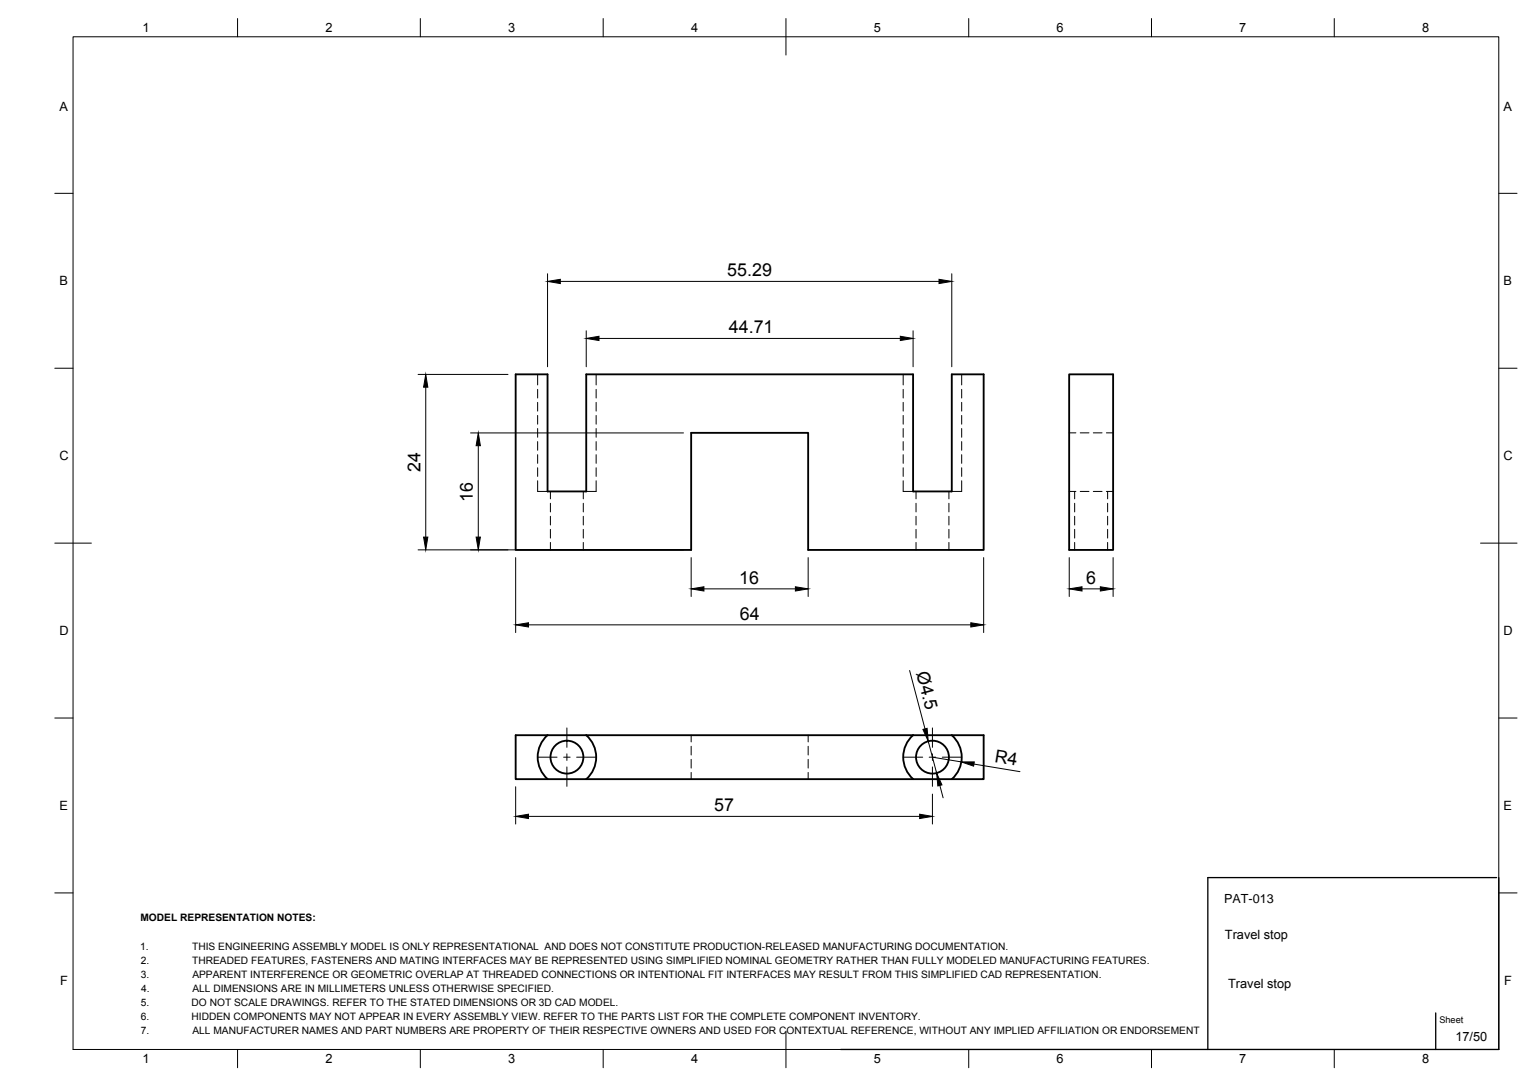
ISO-10303-21;
HEADER;
/* Generated by software containing ST-Developer
 * from STEP Tools, Inc. (www.steptools.com) 
 */

FILE_DESCRIPTION(
/* description */ ('Belt-driven linear axis on 2020 extrusion'),
/* implementation_level */ '2;1');

FILE_NAME(
/* name */ 'Travel stop.step',
/* time_stamp */ '2026-10-28T03:26:09-07:00',
/* author */ (''),
/* organization */ (''),
/* preprocessor_version */ 'ST-DEVELOPER v20.2',
/* originating_system */ 'Autodesk Translation Framework v15.17.0.0',
/* authorisation */ '');

FILE_SCHEMA (('AUTOMOTIVE_DESIGN { 1 0 10303 214 3 1 1 }'));
ENDSEC;

DATA;
#10=MECHANICAL_DESIGN_GEOMETRIC_PRESENTATION_REPRESENTATION('',(#624),#20096);
#530=SHAPE_REPRESENTATION_RELATIONSHIP('SRR','None',#20326,#576);
#576=ADVANCED_BREP_SHAPE_REPRESENTATION('',(#680),#20057);
#624=STYLED_ITEM('',(#20636),#680);
#680=MANIFOLD_SOLID_BREP('Body1',#10937);
#796=FACE_BOUND('',#2127,.T.);
#797=FACE_BOUND('',#2131,.T.);
#798=FACE_BOUND('',#2143,.T.);
#799=FACE_BOUND('',#2145,.T.);
#977=PLANE('',#11857);
#978=PLANE('',#11865);
#979=PLANE('',#11867);
#980=PLANE('',#11868);
#981=PLANE('',#11869);
#982=PLANE('',#11870);
#983=PLANE('',#11875);
#984=PLANE('',#11876);
#985=PLANE('',#11877);
#986=PLANE('',#11878);
#987=PLANE('',#11879);
#988=PLANE('',#11880);
#989=PLANE('',#11881);
#990=PLANE('',#11882);
#1424=FACE_OUTER_BOUND('',#2124,.T.);
#1425=FACE_OUTER_BOUND('',#2125,.T.);
#1426=FACE_OUTER_BOUND('',#2126,.T.);
#1427=FACE_OUTER_BOUND('',#2128,.T.);
#1428=FACE_OUTER_BOUND('',#2129,.T.);
#1429=FACE_OUTER_BOUND('',#2130,.T.);
#1430=FACE_OUTER_BOUND('',#2132,.T.);
#1431=FACE_OUTER_BOUND('',#2133,.T.);
#1432=FACE_OUTER_BOUND('',#2134,.T.);
#1433=FACE_OUTER_BOUND('',#2135,.T.);
#1434=FACE_OUTER_BOUND('',#2136,.T.);
#1435=FACE_OUTER_BOUND('',#2137,.T.);
#1436=FACE_OUTER_BOUND('',#2138,.T.);
#1437=FACE_OUTER_BOUND('',#2139,.T.);
#1438=FACE_OUTER_BOUND('',#2140,.T.);
#1439=FACE_OUTER_BOUND('',#2141,.T.);
#1440=FACE_OUTER_BOUND('',#2142,.T.);
#1441=FACE_OUTER_BOUND('',#2144,.T.);
#1442=FACE_OUTER_BOUND('',#2146,.T.);
#1443=FACE_OUTER_BOUND('',#2147,.T.);
#2124=EDGE_LOOP('',(#8009,#8010,#8011,#8012));
#2125=EDGE_LOOP('',(#8013,#8014,#8015,#8016));
#2126=EDGE_LOOP('',(#8017,#8018,#8019,#8020));
#2127=EDGE_LOOP('',(#8021));
#2128=EDGE_LOOP('',(#8022,#8023,#8024,#8025));
#2129=EDGE_LOOP('',(#8026,#8027,#8028,#8029));
#2130=EDGE_LOOP('',(#8030,#8031,#8032,#8033));
#2131=EDGE_LOOP('',(#8034));
#2132=EDGE_LOOP('',(#8035,#8036,#8037,#8038,#8039,#8040,#8041,#8042,#8043,
#8044,#8045,#8046,#8047,#8048,#8049,#8050));
#2133=EDGE_LOOP('',(#8051,#8052,#8053,#8054));
#2134=EDGE_LOOP('',(#8055,#8056,#8057,#8058));
#2135=EDGE_LOOP('',(#8059,#8060,#8061,#8062));
#2136=EDGE_LOOP('',(#8063,#8064,#8065,#8066));
#2137=EDGE_LOOP('',(#8067,#8068,#8069,#8070));
#2138=EDGE_LOOP('',(#8071,#8072,#8073,#8074));
#2139=EDGE_LOOP('',(#8075,#8076,#8077,#8078));
#2140=EDGE_LOOP('',(#8079,#8080,#8081,#8082));
#2141=EDGE_LOOP('',(#8083,#8084,#8085,#8086,#8087,#8088,#8089,#8090,#8091,
#8092,#8093,#8094,#8095,#8096,#8097,#8098));
#2142=EDGE_LOOP('',(#8099,#8100,#8101,#8102));
#2143=EDGE_LOOP('',(#8103));
#2144=EDGE_LOOP('',(#8104,#8105,#8106,#8107));
#2145=EDGE_LOOP('',(#8108));
#2146=EDGE_LOOP('',(#8109,#8110,#8111,#8112));
#2147=EDGE_LOOP('',(#8113,#8114,#8115,#8116));
#2871=LINE('',#17054,#3728);
#2872=LINE('',#17058,#3729);
#2873=LINE('',#17063,#3730);
#2874=LINE('',#17067,#3731);
#2875=LINE('',#17070,#3732);
#2876=LINE('',#17071,#3733);
#2877=LINE('',#17077,#3734);
#2878=LINE('',#17081,#3735);
#2879=LINE('',#17086,#3736);
#2880=LINE('',#17090,#3737);
#2881=LINE('',#17093,#3738);
#2882=LINE('',#17094,#3739);
#2883=LINE('',#17099,#3740);
#2884=LINE('',#17101,#3741);
#2885=LINE('',#17103,#3742);
#2886=LINE('',#17105,#3743);
#2887=LINE('',#17107,#3744);
#2888=LINE('',#17109,#3745);
#2889=LINE('',#17111,#3746);
#2890=LINE('',#17113,#3747);
#2891=LINE('',#17114,#3748);
#2892=LINE('',#17115,#3749);
#2893=LINE('',#17118,#3750);
#2894=LINE('',#17119,#3751);
#2895=LINE('',#17122,#3752);
#2896=LINE('',#17123,#3753);
#2897=LINE('',#17125,#3754);
#2898=LINE('',#17129,#3755);
#2899=LINE('',#17133,#3756);
#2900=LINE('',#17136,#3757);
#2901=LINE('',#17138,#3758);
#2902=LINE('',#17139,#3759);
#2903=LINE('',#17142,#3760);
#2904=LINE('',#17144,#3761);
#2905=LINE('',#17145,#3762);
#2906=LINE('',#17147,#3763);
#2907=LINE('',#17150,#3764);
#2908=LINE('',#17151,#3765);
#2909=LINE('',#17153,#3766);
#2910=LINE('',#17154,#3767);
#2911=LINE('',#17156,#3768);
#2912=LINE('',#17158,#3769);
#3728=VECTOR('',#13715,1.);
#3729=VECTOR('',#13718,1.);
#3730=VECTOR('',#13723,1.);
#3731=VECTOR('',#13726,1.);
#3732=VECTOR('',#13731,1.);
#3733=VECTOR('',#13732,1.);
#3734=VECTOR('',#13737,1.);
#3735=VECTOR('',#13740,1.);
#3736=VECTOR('',#13745,1.);
#3737=VECTOR('',#13748,1.);
#3738=VECTOR('',#13753,1.);
#3739=VECTOR('',#13754,1.);
#3740=VECTOR('',#13759,1.);
#3741=VECTOR('',#13760,1.);
#3742=VECTOR('',#13761,1.);
#3743=VECTOR('',#13762,1.);
#3744=VECTOR('',#13763,1.);
#3745=VECTOR('',#13764,1.);
#3746=VECTOR('',#13765,1.);
#3747=VECTOR('',#13766,1.);
#3748=VECTOR('',#13767,1.);
#3749=VECTOR('',#13768,1.);
#3750=VECTOR('',#13771,1.);
#3751=VECTOR('',#13772,1.);
#3752=VECTOR('',#13775,1.);
#3753=VECTOR('',#13776,1.);
#3754=VECTOR('',#13779,1.);
#3755=VECTOR('',#13784,0.225);
#3756=VECTOR('',#13789,0.225);
#3757=VECTOR('',#13792,1.);
#3758=VECTOR('',#13793,1.);
#3759=VECTOR('',#13794,1.);
#3760=VECTOR('',#13797,1.);
#3761=VECTOR('',#13798,1.);
#3762=VECTOR('',#13799,1.);
#3763=VECTOR('',#13802,1.);
#3764=VECTOR('',#13805,1.);
#3765=VECTOR('',#13806,1.);
#3766=VECTOR('',#13807,1.);
#3767=VECTOR('',#13808,1.);
#3768=VECTOR('',#13811,1.);
#3769=VECTOR('',#13814,1.);
#4551=CIRCLE('',#11852,0.4);
#4552=CIRCLE('',#11853,0.4);
#4553=CIRCLE('',#11855,0.4);
#4554=CIRCLE('',#11856,0.4);
#4555=CIRCLE('',#11858,0.225);
#4556=CIRCLE('',#11860,0.4);
#4557=CIRCLE('',#11861,0.4);
#4558=CIRCLE('',#11863,0.4);
#4559=CIRCLE('',#11864,0.4);
#4560=CIRCLE('',#11866,0.225);
#4561=CIRCLE('',#11872,0.225);
#4562=CIRCLE('',#11874,0.225);
#5144=VERTEX_POINT('',#17052);
#5145=VERTEX_POINT('',#17053);
#5146=VERTEX_POINT('',#17055);
#5147=VERTEX_POINT('',#17057);
#5148=VERTEX_POINT('',#17061);
#5149=VERTEX_POINT('',#17062);
#5150=VERTEX_POINT('',#17064);
#5151=VERTEX_POINT('',#17066);
#5152=VERTEX_POINT('',#17072);
#5153=VERTEX_POINT('',#17075);
#5154=VERTEX_POINT('',#17076);
#5155=VERTEX_POINT('',#17078);
#5156=VERTEX_POINT('',#17080);
#5157=VERTEX_POINT('',#17084);
#5158=VERTEX_POINT('',#17085);
#5159=VERTEX_POINT('',#17087);
#5160=VERTEX_POINT('',#17089);
#5161=VERTEX_POINT('',#17095);
#5162=VERTEX_POINT('',#17098);
#5163=VERTEX_POINT('',#17100);
#5164=VERTEX_POINT('',#17102);
#5165=VERTEX_POINT('',#17104);
#5166=VERTEX_POINT('',#17106);
#5167=VERTEX_POINT('',#17108);
#5168=VERTEX_POINT('',#17110);
#5169=VERTEX_POINT('',#17112);
#5170=VERTEX_POINT('',#17117);
#5171=VERTEX_POINT('',#17121);
#5172=VERTEX_POINT('',#17127);
#5173=VERTEX_POINT('',#17131);
#5174=VERTEX_POINT('',#17135);
#5175=VERTEX_POINT('',#17137);
#5176=VERTEX_POINT('',#17141);
#5177=VERTEX_POINT('',#17143);
#5178=VERTEX_POINT('',#17149);
#5179=VERTEX_POINT('',#17152);
#6219=EDGE_CURVE('',#5144,#5145,#2871,.T.);
#6220=EDGE_CURVE('',#5146,#5144,#4551,.T.);
#6221=EDGE_CURVE('',#5147,#5146,#2872,.T.);
#6222=EDGE_CURVE('',#5145,#5147,#4552,.T.);
#6223=EDGE_CURVE('',#5148,#5149,#2873,.T.);
#6224=EDGE_CURVE('',#5150,#5148,#4553,.T.);
#6225=EDGE_CURVE('',#5151,#5150,#2874,.T.);
#6226=EDGE_CURVE('',#5149,#5151,#4554,.T.);
#6227=EDGE_CURVE('',#5145,#5148,#2875,.T.);
#6228=EDGE_CURVE('',#5150,#5147,#2876,.T.);
#6229=EDGE_CURVE('',#5152,#5152,#4555,.T.);
#6230=EDGE_CURVE('',#5153,#5154,#2877,.T.);
#6231=EDGE_CURVE('',#5155,#5153,#4556,.T.);
#6232=EDGE_CURVE('',#5156,#5155,#2878,.T.);
#6233=EDGE_CURVE('',#5154,#5156,#4557,.T.);
#6234=EDGE_CURVE('',#5157,#5158,#2879,.T.);
#6235=EDGE_CURVE('',#5159,#5157,#4558,.T.);
#6236=EDGE_CURVE('',#5160,#5159,#2880,.T.);
#6237=EDGE_CURVE('',#5158,#5160,#4559,.T.);
#6238=EDGE_CURVE('',#5154,#5157,#2881,.T.);
#6239=EDGE_CURVE('',#5159,#5156,#2882,.T.);
#6240=EDGE_CURVE('',#5161,#5161,#4560,.T.);
#6241=EDGE_CURVE('',#5162,#5146,#2883,.T.);
#6242=EDGE_CURVE('',#5163,#5162,#2884,.T.);
#6243=EDGE_CURVE('',#5163,#5164,#2885,.T.);
#6244=EDGE_CURVE('',#5164,#5165,#2886,.T.);
#6245=EDGE_CURVE('',#5165,#5166,#2887,.T.);
#6246=EDGE_CURVE('',#5166,#5167,#2888,.T.);
#6247=EDGE_CURVE('',#5167,#5168,#2889,.T.);
#6248=EDGE_CURVE('',#5168,#5169,#2890,.T.);
#6249=EDGE_CURVE('',#5160,#5169,#2891,.T.);
#6250=EDGE_CURVE('',#5151,#5155,#2892,.T.);
#6251=EDGE_CURVE('',#5169,#5170,#2893,.T.);
#6252=EDGE_CURVE('',#5170,#5158,#2894,.T.);
#6253=EDGE_CURVE('',#5144,#5171,#2895,.T.);
#6254=EDGE_CURVE('',#5171,#5162,#2896,.T.);
#6255=EDGE_CURVE('',#5153,#5149,#2897,.T.);
#6256=EDGE_CURVE('',#5172,#5172,#4561,.T.);
#6257=EDGE_CURVE('',#5172,#5152,#2898,.T.);
#6258=EDGE_CURVE('',#5173,#5173,#4562,.T.);
#6259=EDGE_CURVE('',#5173,#5161,#2899,.T.);
#6260=EDGE_CURVE('',#5166,#5174,#2900,.T.);
#6261=EDGE_CURVE('',#5175,#5174,#2901,.T.);
#6262=EDGE_CURVE('',#5167,#5175,#2902,.T.);
#6263=EDGE_CURVE('',#5176,#5164,#2903,.T.);
#6264=EDGE_CURVE('',#5177,#5176,#2904,.T.);
#6265=EDGE_CURVE('',#5177,#5165,#2905,.T.);
#6266=EDGE_CURVE('',#5174,#5177,#2906,.T.);
#6267=EDGE_CURVE('',#5178,#5170,#2907,.T.);
#6268=EDGE_CURVE('',#5178,#5175,#2908,.T.);
#6269=EDGE_CURVE('',#5176,#5179,#2909,.T.);
#6270=EDGE_CURVE('',#5179,#5171,#2910,.T.);
#6271=EDGE_CURVE('',#5179,#5163,#2911,.T.);
#6272=EDGE_CURVE('',#5168,#5178,#2912,.T.);
#8009=ORIENTED_EDGE('',*,*,#6219,.F.);
#8010=ORIENTED_EDGE('',*,*,#6220,.F.);
#8011=ORIENTED_EDGE('',*,*,#6221,.F.);
#8012=ORIENTED_EDGE('',*,*,#6222,.F.);
#8013=ORIENTED_EDGE('',*,*,#6223,.F.);
#8014=ORIENTED_EDGE('',*,*,#6224,.F.);
#8015=ORIENTED_EDGE('',*,*,#6225,.F.);
#8016=ORIENTED_EDGE('',*,*,#6226,.F.);
#8017=ORIENTED_EDGE('',*,*,#6227,.F.);
#8018=ORIENTED_EDGE('',*,*,#6222,.T.);
#8019=ORIENTED_EDGE('',*,*,#6228,.F.);
#8020=ORIENTED_EDGE('',*,*,#6224,.T.);
#8021=ORIENTED_EDGE('',*,*,#6229,.F.);
#8022=ORIENTED_EDGE('',*,*,#6230,.F.);
#8023=ORIENTED_EDGE('',*,*,#6231,.F.);
#8024=ORIENTED_EDGE('',*,*,#6232,.F.);
#8025=ORIENTED_EDGE('',*,*,#6233,.F.);
#8026=ORIENTED_EDGE('',*,*,#6234,.F.);
#8027=ORIENTED_EDGE('',*,*,#6235,.F.);
#8028=ORIENTED_EDGE('',*,*,#6236,.F.);
#8029=ORIENTED_EDGE('',*,*,#6237,.F.);
#8030=ORIENTED_EDGE('',*,*,#6238,.F.);
#8031=ORIENTED_EDGE('',*,*,#6233,.T.);
#8032=ORIENTED_EDGE('',*,*,#6239,.F.);
#8033=ORIENTED_EDGE('',*,*,#6235,.T.);
#8034=ORIENTED_EDGE('',*,*,#6240,.F.);
#8035=ORIENTED_EDGE('',*,*,#6225,.T.);
#8036=ORIENTED_EDGE('',*,*,#6228,.T.);
#8037=ORIENTED_EDGE('',*,*,#6221,.T.);
#8038=ORIENTED_EDGE('',*,*,#6241,.F.);
#8039=ORIENTED_EDGE('',*,*,#6242,.F.);
#8040=ORIENTED_EDGE('',*,*,#6243,.T.);
#8041=ORIENTED_EDGE('',*,*,#6244,.T.);
#8042=ORIENTED_EDGE('',*,*,#6245,.T.);
#8043=ORIENTED_EDGE('',*,*,#6246,.T.);
#8044=ORIENTED_EDGE('',*,*,#6247,.T.);
#8045=ORIENTED_EDGE('',*,*,#6248,.T.);
#8046=ORIENTED_EDGE('',*,*,#6249,.F.);
#8047=ORIENTED_EDGE('',*,*,#6236,.T.);
#8048=ORIENTED_EDGE('',*,*,#6239,.T.);
#8049=ORIENTED_EDGE('',*,*,#6232,.T.);
#8050=ORIENTED_EDGE('',*,*,#6250,.F.);
#8051=ORIENTED_EDGE('',*,*,#6237,.T.);
#8052=ORIENTED_EDGE('',*,*,#6249,.T.);
#8053=ORIENTED_EDGE('',*,*,#6251,.T.);
#8054=ORIENTED_EDGE('',*,*,#6252,.T.);
#8055=ORIENTED_EDGE('',*,*,#6220,.T.);
#8056=ORIENTED_EDGE('',*,*,#6253,.T.);
#8057=ORIENTED_EDGE('',*,*,#6254,.T.);
#8058=ORIENTED_EDGE('',*,*,#6241,.T.);
#8059=ORIENTED_EDGE('',*,*,#6226,.T.);
#8060=ORIENTED_EDGE('',*,*,#6250,.T.);
#8061=ORIENTED_EDGE('',*,*,#6231,.T.);
#8062=ORIENTED_EDGE('',*,*,#6255,.T.);
#8063=ORIENTED_EDGE('',*,*,#6256,.F.);
#8064=ORIENTED_EDGE('',*,*,#6257,.T.);
#8065=ORIENTED_EDGE('',*,*,#6229,.T.);
#8066=ORIENTED_EDGE('',*,*,#6257,.F.);
#8067=ORIENTED_EDGE('',*,*,#6258,.F.);
#8068=ORIENTED_EDGE('',*,*,#6259,.T.);
#8069=ORIENTED_EDGE('',*,*,#6240,.T.);
#8070=ORIENTED_EDGE('',*,*,#6259,.F.);
#8071=ORIENTED_EDGE('',*,*,#6246,.F.);
#8072=ORIENTED_EDGE('',*,*,#6260,.T.);
#8073=ORIENTED_EDGE('',*,*,#6261,.F.);
#8074=ORIENTED_EDGE('',*,*,#6262,.F.);
#8075=ORIENTED_EDGE('',*,*,#6244,.F.);
#8076=ORIENTED_EDGE('',*,*,#6263,.F.);
#8077=ORIENTED_EDGE('',*,*,#6264,.F.);
#8078=ORIENTED_EDGE('',*,*,#6265,.T.);
#8079=ORIENTED_EDGE('',*,*,#6245,.F.);
#8080=ORIENTED_EDGE('',*,*,#6265,.F.);
#8081=ORIENTED_EDGE('',*,*,#6266,.F.);
#8082=ORIENTED_EDGE('',*,*,#6260,.F.);
#8083=ORIENTED_EDGE('',*,*,#6223,.T.);
#8084=ORIENTED_EDGE('',*,*,#6255,.F.);
#8085=ORIENTED_EDGE('',*,*,#6230,.T.);
#8086=ORIENTED_EDGE('',*,*,#6238,.T.);
#8087=ORIENTED_EDGE('',*,*,#6234,.T.);
#8088=ORIENTED_EDGE('',*,*,#6252,.F.);
#8089=ORIENTED_EDGE('',*,*,#6267,.F.);
#8090=ORIENTED_EDGE('',*,*,#6268,.T.);
#8091=ORIENTED_EDGE('',*,*,#6261,.T.);
#8092=ORIENTED_EDGE('',*,*,#6266,.T.);
#8093=ORIENTED_EDGE('',*,*,#6264,.T.);
#8094=ORIENTED_EDGE('',*,*,#6269,.T.);
#8095=ORIENTED_EDGE('',*,*,#6270,.T.);
#8096=ORIENTED_EDGE('',*,*,#6253,.F.);
#8097=ORIENTED_EDGE('',*,*,#6219,.T.);
#8098=ORIENTED_EDGE('',*,*,#6227,.T.);
#8099=ORIENTED_EDGE('',*,*,#6263,.T.);
#8100=ORIENTED_EDGE('',*,*,#6243,.F.);
#8101=ORIENTED_EDGE('',*,*,#6271,.F.);
#8102=ORIENTED_EDGE('',*,*,#6269,.F.);
#8103=ORIENTED_EDGE('',*,*,#6256,.T.);
#8104=ORIENTED_EDGE('',*,*,#6262,.T.);
#8105=ORIENTED_EDGE('',*,*,#6268,.F.);
#8106=ORIENTED_EDGE('',*,*,#6272,.F.);
#8107=ORIENTED_EDGE('',*,*,#6247,.F.);
#8108=ORIENTED_EDGE('',*,*,#6258,.T.);
#8109=ORIENTED_EDGE('',*,*,#6272,.T.);
#8110=ORIENTED_EDGE('',*,*,#6267,.T.);
#8111=ORIENTED_EDGE('',*,*,#6251,.F.);
#8112=ORIENTED_EDGE('',*,*,#6248,.F.);
#8113=ORIENTED_EDGE('',*,*,#6271,.T.);
#8114=ORIENTED_EDGE('',*,*,#6242,.T.);
#8115=ORIENTED_EDGE('',*,*,#6254,.F.);
#8116=ORIENTED_EDGE('',*,*,#6270,.F.);
#10163=CYLINDRICAL_SURFACE('',#11851,0.4);
#10164=CYLINDRICAL_SURFACE('',#11854,0.4);
#10165=CYLINDRICAL_SURFACE('',#11859,0.4);
#10166=CYLINDRICAL_SURFACE('',#11862,0.4);
#10167=CYLINDRICAL_SURFACE('',#11871,0.225);
#10168=CYLINDRICAL_SURFACE('',#11873,0.225);
#10475=ADVANCED_FACE('',(#1424),#10163,.F.);
#10476=ADVANCED_FACE('',(#1425),#10164,.F.);
#10477=ADVANCED_FACE('',(#1426,#796),#977,.T.);
#10478=ADVANCED_FACE('',(#1427),#10165,.F.);
#10479=ADVANCED_FACE('',(#1428),#10166,.F.);
#10480=ADVANCED_FACE('',(#1429,#797),#978,.T.);
#10481=ADVANCED_FACE('',(#1430),#979,.T.);
#10482=ADVANCED_FACE('',(#1431),#980,.T.);
#10483=ADVANCED_FACE('',(#1432),#981,.T.);
#10484=ADVANCED_FACE('',(#1433),#982,.T.);
#10485=ADVANCED_FACE('',(#1434),#10167,.F.);
#10486=ADVANCED_FACE('',(#1435),#10168,.F.);
#10487=ADVANCED_FACE('',(#1436),#983,.F.);
#10488=ADVANCED_FACE('',(#1437),#984,.F.);
#10489=ADVANCED_FACE('',(#1438),#985,.F.);
#10490=ADVANCED_FACE('',(#1439),#986,.T.);
#10491=ADVANCED_FACE('',(#1440,#798),#987,.F.);
#10492=ADVANCED_FACE('',(#1441,#799),#988,.F.);
#10493=ADVANCED_FACE('',(#1442),#989,.T.);
#10494=ADVANCED_FACE('',(#1443),#990,.T.);
#10937=CLOSED_SHELL('',(#10475,#10476,#10477,#10478,#10479,#10480,#10481,
#10482,#10483,#10484,#10485,#10486,#10487,#10488,#10489,#10490,#10491,#10492,
#10493,#10494));
#11850=AXIS2_PLACEMENT_3D('',#17050,#13711,#13712);
#11851=AXIS2_PLACEMENT_3D('',#17051,#13713,#13714);
#11852=AXIS2_PLACEMENT_3D('',#17056,#13716,#13717);
#11853=AXIS2_PLACEMENT_3D('',#17059,#13719,#13720);
#11854=AXIS2_PLACEMENT_3D('',#17060,#13721,#13722);
#11855=AXIS2_PLACEMENT_3D('',#17065,#13724,#13725);
#11856=AXIS2_PLACEMENT_3D('',#17068,#13727,#13728);
#11857=AXIS2_PLACEMENT_3D('',#17069,#13729,#13730);
#11858=AXIS2_PLACEMENT_3D('',#17073,#13733,#13734);
#11859=AXIS2_PLACEMENT_3D('',#17074,#13735,#13736);
#11860=AXIS2_PLACEMENT_3D('',#17079,#13738,#13739);
#11861=AXIS2_PLACEMENT_3D('',#17082,#13741,#13742);
#11862=AXIS2_PLACEMENT_3D('',#17083,#13743,#13744);
#11863=AXIS2_PLACEMENT_3D('',#17088,#13746,#13747);
#11864=AXIS2_PLACEMENT_3D('',#17091,#13749,#13750);
#11865=AXIS2_PLACEMENT_3D('',#17092,#13751,#13752);
#11866=AXIS2_PLACEMENT_3D('',#17096,#13755,#13756);
#11867=AXIS2_PLACEMENT_3D('',#17097,#13757,#13758);
#11868=AXIS2_PLACEMENT_3D('',#17116,#13769,#13770);
#11869=AXIS2_PLACEMENT_3D('',#17120,#13773,#13774);
#11870=AXIS2_PLACEMENT_3D('',#17124,#13777,#13778);
#11871=AXIS2_PLACEMENT_3D('',#17126,#13780,#13781);
#11872=AXIS2_PLACEMENT_3D('',#17128,#13782,#13783);
#11873=AXIS2_PLACEMENT_3D('',#17130,#13785,#13786);
#11874=AXIS2_PLACEMENT_3D('',#17132,#13787,#13788);
#11875=AXIS2_PLACEMENT_3D('',#17134,#13790,#13791);
#11876=AXIS2_PLACEMENT_3D('',#17140,#13795,#13796);
#11877=AXIS2_PLACEMENT_3D('',#17146,#13800,#13801);
#11878=AXIS2_PLACEMENT_3D('',#17148,#13803,#13804);
#11879=AXIS2_PLACEMENT_3D('',#17155,#13809,#13810);
#11880=AXIS2_PLACEMENT_3D('',#17157,#13812,#13813);
#11881=AXIS2_PLACEMENT_3D('',#17159,#13815,#13816);
#11882=AXIS2_PLACEMENT_3D('',#17160,#13817,#13818);
#13711=DIRECTION('axis',(0.,0.,1.));
#13712=DIRECTION('refdir',(1.,0.,0.));
#13713=DIRECTION('center_axis',(0.,0.,1.));
#13714=DIRECTION('ref_axis',(1.,0.,0.));
#13715=DIRECTION('',(0.,0.,-1.));
#13716=DIRECTION('center_axis',(0.,0.,-1.));
#13717=DIRECTION('ref_axis',(1.,0.,0.));
#13718=DIRECTION('',(0.,0.,1.));
#13719=DIRECTION('center_axis',(0.,0.,1.));
#13720=DIRECTION('ref_axis',(1.,0.,0.));
#13721=DIRECTION('center_axis',(0.,0.,1.));
#13722=DIRECTION('ref_axis',(1.,0.,0.));
#13723=DIRECTION('',(0.,0.,1.));
#13724=DIRECTION('center_axis',(0.,0.,1.));
#13725=DIRECTION('ref_axis',(1.,0.,0.));
#13726=DIRECTION('',(0.,0.,-1.));
#13727=DIRECTION('center_axis',(0.,0.,-1.));
#13728=DIRECTION('ref_axis',(1.,0.,0.));
#13729=DIRECTION('center_axis',(0.,0.,1.));
#13730=DIRECTION('ref_axis',(1.,0.,0.));
#13731=DIRECTION('',(0.,1.,0.));
#13732=DIRECTION('',(0.,-1.,0.));
#13733=DIRECTION('center_axis',(0.,0.,1.));
#13734=DIRECTION('ref_axis',(1.,0.,0.));
#13735=DIRECTION('center_axis',(0.,0.,1.));
#13736=DIRECTION('ref_axis',(1.,0.,0.));
#13737=DIRECTION('',(0.,0.,-1.));
#13738=DIRECTION('center_axis',(0.,0.,-1.));
#13739=DIRECTION('ref_axis',(1.,0.,0.));
#13740=DIRECTION('',(0.,0.,1.));
#13741=DIRECTION('center_axis',(0.,0.,1.));
#13742=DIRECTION('ref_axis',(1.,0.,0.));
#13743=DIRECTION('center_axis',(0.,0.,1.));
#13744=DIRECTION('ref_axis',(1.,0.,0.));
#13745=DIRECTION('',(0.,0.,1.));
#13746=DIRECTION('center_axis',(0.,0.,1.));
#13747=DIRECTION('ref_axis',(1.,0.,0.));
#13748=DIRECTION('',(0.,0.,-1.));
#13749=DIRECTION('center_axis',(0.,0.,-1.));
#13750=DIRECTION('ref_axis',(1.,0.,0.));
#13751=DIRECTION('center_axis',(0.,0.,1.));
#13752=DIRECTION('ref_axis',(1.,0.,0.));
#13753=DIRECTION('',(0.,1.,0.));
#13754=DIRECTION('',(0.,-1.,0.));
#13755=DIRECTION('center_axis',(0.,0.,1.));
#13756=DIRECTION('ref_axis',(1.,0.,0.));
#13757=DIRECTION('center_axis',(1.,0.,0.));
#13758=DIRECTION('ref_axis',(0.,1.,0.));
#13759=DIRECTION('',(0.,1.,0.));
#13760=DIRECTION('',(0.,0.,1.));
#13761=DIRECTION('',(0.,1.,0.));
#13762=DIRECTION('',(0.,0.,1.));
#13763=DIRECTION('',(0.,1.,0.));
#13764=DIRECTION('',(0.,0.,-1.));
#13765=DIRECTION('',(0.,1.,0.));
#13766=DIRECTION('',(0.,0.,1.));
#13767=DIRECTION('',(0.,1.,0.));
#13768=DIRECTION('',(0.,1.,0.));
#13769=DIRECTION('center_axis',(0.,0.,1.));
#13770=DIRECTION('ref_axis',(1.,0.,0.));
#13771=DIRECTION('',(-1.,0.,0.));
#13772=DIRECTION('',(0.,-1.,0.));
#13773=DIRECTION('center_axis',(0.,0.,1.));
#13774=DIRECTION('ref_axis',(1.,0.,0.));
#13775=DIRECTION('',(0.,-1.,0.));
#13776=DIRECTION('',(1.,0.,0.));
#13777=DIRECTION('center_axis',(0.,0.,1.));
#13778=DIRECTION('ref_axis',(1.,0.,0.));
#13779=DIRECTION('',(0.,-1.,0.));
#13780=DIRECTION('center_axis',(0.,0.,1.));
#13781=DIRECTION('ref_axis',(1.,0.,0.));
#13782=DIRECTION('center_axis',(0.,0.,1.));
#13783=DIRECTION('ref_axis',(1.,0.,0.));
#13784=DIRECTION('',(0.,0.,1.));
#13785=DIRECTION('center_axis',(0.,0.,1.));
#13786=DIRECTION('ref_axis',(1.,0.,0.));
#13787=DIRECTION('center_axis',(0.,0.,1.));
#13788=DIRECTION('ref_axis',(1.,0.,0.));
#13789=DIRECTION('',(0.,0.,1.));
#13790=DIRECTION('center_axis',(0.,1.,0.));
#13791=DIRECTION('ref_axis',(-1.,0.,0.));
#13792=DIRECTION('',(-1.,0.,0.));
#13793=DIRECTION('',(0.,0.,1.));
#13794=DIRECTION('',(-1.,0.,0.));
#13795=DIRECTION('center_axis',(0.,-1.,0.));
#13796=DIRECTION('ref_axis',(1.,0.,0.));
#13797=DIRECTION('',(1.,0.,0.));
#13798=DIRECTION('',(0.,0.,-1.));
#13799=DIRECTION('',(1.,0.,0.));
#13800=DIRECTION('center_axis',(0.,0.,1.));
#13801=DIRECTION('ref_axis',(1.,0.,0.));
#13802=DIRECTION('',(0.,-1.,0.));
#13803=DIRECTION('center_axis',(-1.,0.,0.));
#13804=DIRECTION('ref_axis',(0.,-1.,0.));
#13805=DIRECTION('',(0.,0.,1.));
#13806=DIRECTION('',(0.,-1.,0.));
#13807=DIRECTION('',(0.,-1.,0.));
#13808=DIRECTION('',(0.,0.,1.));
#13809=DIRECTION('center_axis',(0.,0.,1.));
#13810=DIRECTION('ref_axis',(1.,0.,0.));
#13811=DIRECTION('',(1.,0.,0.));
#13812=DIRECTION('center_axis',(0.,0.,1.));
#13813=DIRECTION('ref_axis',(1.,0.,0.));
#13814=DIRECTION('',(-1.,0.,0.));
#13815=DIRECTION('center_axis',(0.,1.,0.));
#13816=DIRECTION('ref_axis',(-1.,0.,0.));
#13817=DIRECTION('center_axis',(0.,-1.,0.));
#13818=DIRECTION('ref_axis',(1.,0.,0.));
#17050=CARTESIAN_POINT('',(0.,0.,0.));
#17051=CARTESIAN_POINT('Origin',(5.8,-2.5,0.8));
#17052=CARTESIAN_POINT('',(5.5,-2.76457513110646,2.4));
#17053=CARTESIAN_POINT('',(5.5,-2.76457513110646,0.8));
#17054=CARTESIAN_POINT('',(5.5,-2.76457513110646,0.8));
#17055=CARTESIAN_POINT('',(6.1,-2.76457513110646,2.4));
#17056=CARTESIAN_POINT('Origin',(5.8,-2.5,2.4));
#17057=CARTESIAN_POINT('',(6.1,-2.76457513110646,0.8));
#17058=CARTESIAN_POINT('',(6.1,-2.76457513110646,0.8));
#17059=CARTESIAN_POINT('Origin',(5.8,-2.5,0.8));
#17060=CARTESIAN_POINT('Origin',(5.8,-2.5,0.8));
#17061=CARTESIAN_POINT('',(5.5,-2.23542486889354,0.8));
#17062=CARTESIAN_POINT('',(5.5,-2.23542486889354,2.4));
#17063=CARTESIAN_POINT('',(5.5,-2.23542486889354,0.8));
#17064=CARTESIAN_POINT('',(6.1,-2.23542486889354,0.8));
#17065=CARTESIAN_POINT('Origin',(5.8,-2.5,0.8));
#17066=CARTESIAN_POINT('',(6.1,-2.23542486889354,2.4));
#17067=CARTESIAN_POINT('',(6.1,-2.23542486889354,0.8));
#17068=CARTESIAN_POINT('Origin',(5.8,-2.5,2.4));
#17069=CARTESIAN_POINT('Origin',(5.8,-2.5,0.8));
#17070=CARTESIAN_POINT('',(5.5,0.35,0.8));
#17071=CARTESIAN_POINT('',(6.1,-2.85,0.8));
#17072=CARTESIAN_POINT('',(5.575,-2.5,0.8));
#17073=CARTESIAN_POINT('Origin',(5.8,-2.5,0.8));
#17074=CARTESIAN_POINT('Origin',(5.8,2.5,0.8));
#17075=CARTESIAN_POINT('',(5.5,2.23542486889354,2.4));
#17076=CARTESIAN_POINT('',(5.5,2.23542486889354,0.8));
#17077=CARTESIAN_POINT('',(5.5,2.23542486889354,0.8));
#17078=CARTESIAN_POINT('',(6.1,2.23542486889354,2.4));
#17079=CARTESIAN_POINT('Origin',(5.8,2.5,2.4));
#17080=CARTESIAN_POINT('',(6.1,2.23542486889354,0.8));
#17081=CARTESIAN_POINT('',(6.1,2.23542486889354,0.8));
#17082=CARTESIAN_POINT('Origin',(5.8,2.5,0.8));
#17083=CARTESIAN_POINT('Origin',(5.8,2.5,0.8));
#17084=CARTESIAN_POINT('',(5.5,2.76457513110646,0.8));
#17085=CARTESIAN_POINT('',(5.5,2.76457513110646,2.4));
#17086=CARTESIAN_POINT('',(5.5,2.76457513110646,0.8));
#17087=CARTESIAN_POINT('',(6.1,2.76457513110646,0.8));
#17088=CARTESIAN_POINT('Origin',(5.8,2.5,0.8));
#17089=CARTESIAN_POINT('',(6.1,2.76457513110646,2.4));
#17090=CARTESIAN_POINT('',(6.1,2.76457513110646,0.8));
#17091=CARTESIAN_POINT('Origin',(5.8,2.5,2.4));
#17092=CARTESIAN_POINT('Origin',(5.8,2.5,0.8));
#17093=CARTESIAN_POINT('',(5.5,2.85,0.8));
#17094=CARTESIAN_POINT('',(6.1,-0.35,0.8));
#17095=CARTESIAN_POINT('',(5.575,2.5,0.8));
#17096=CARTESIAN_POINT('Origin',(5.8,2.5,0.8));
#17097=CARTESIAN_POINT('Origin',(6.1,-3.2,0.));
#17098=CARTESIAN_POINT('',(6.1,-3.2,2.4));
#17099=CARTESIAN_POINT('',(6.1,-3.2,2.4));
#17100=CARTESIAN_POINT('',(6.1,-3.2,0.));
#17101=CARTESIAN_POINT('',(6.1,-3.2,0.));
#17102=CARTESIAN_POINT('',(6.1,-0.8,0.));
#17103=CARTESIAN_POINT('',(6.1,-3.2,0.));
#17104=CARTESIAN_POINT('',(6.1,-0.8,1.6));
#17105=CARTESIAN_POINT('',(6.1,-0.8,-0.05));
#17106=CARTESIAN_POINT('',(6.1,0.8,1.6));
#17107=CARTESIAN_POINT('',(6.1,-1.6,1.6));
#17108=CARTESIAN_POINT('',(6.1,0.8,0.));
#17109=CARTESIAN_POINT('',(6.1,0.8,-0.05));
#17110=CARTESIAN_POINT('',(6.1,3.2,0.));
#17111=CARTESIAN_POINT('',(6.1,-3.2,0.));
#17112=CARTESIAN_POINT('',(6.1,3.2,2.4));
#17113=CARTESIAN_POINT('',(6.1,3.2,0.));
#17114=CARTESIAN_POINT('',(6.1,-3.2,2.4));
#17115=CARTESIAN_POINT('',(6.1,-3.2,2.4));
#17116=CARTESIAN_POINT('Origin',(5.8,0.,2.4));
#17117=CARTESIAN_POINT('',(5.5,3.2,2.4));
#17118=CARTESIAN_POINT('',(6.1,3.2,2.4));
#17119=CARTESIAN_POINT('',(5.5,3.2,2.4));
#17120=CARTESIAN_POINT('Origin',(5.8,0.,2.4));
#17121=CARTESIAN_POINT('',(5.5,-3.2,2.4));
#17122=CARTESIAN_POINT('',(5.5,3.2,2.4));
#17123=CARTESIAN_POINT('',(5.5,-3.2,2.4));
#17124=CARTESIAN_POINT('Origin',(5.8,0.,2.4));
#17125=CARTESIAN_POINT('',(5.5,3.2,2.4));
#17126=CARTESIAN_POINT('Origin',(5.8,-2.5,-0.1));
#17127=CARTESIAN_POINT('',(5.575,-2.5,0.));
#17128=CARTESIAN_POINT('Origin',(5.8,-2.5,0.));
#17129=CARTESIAN_POINT('',(5.575,-2.5,-0.1));
#17130=CARTESIAN_POINT('Origin',(5.8,2.5,-0.1));
#17131=CARTESIAN_POINT('',(5.575,2.5,0.));
#17132=CARTESIAN_POINT('Origin',(5.8,2.5,0.));
#17133=CARTESIAN_POINT('',(5.575,2.5,-0.1));
#17134=CARTESIAN_POINT('Origin',(6.2,0.8,-0.1));
#17135=CARTESIAN_POINT('',(5.5,0.8,1.6));
#17136=CARTESIAN_POINT('',(6.2,0.8,1.6));
#17137=CARTESIAN_POINT('',(5.5,0.8,0.));
#17138=CARTESIAN_POINT('',(5.5,0.8,-0.05));
#17139=CARTESIAN_POINT('',(6.,0.8,0.));
#17140=CARTESIAN_POINT('Origin',(5.4,-0.8,-0.1));
#17141=CARTESIAN_POINT('',(5.5,-0.8,0.));
#17142=CARTESIAN_POINT('',(5.6,-0.8,0.));
#17143=CARTESIAN_POINT('',(5.5,-0.8,1.6));
#17144=CARTESIAN_POINT('',(5.5,-0.8,-0.05));
#17145=CARTESIAN_POINT('',(5.4,-0.8,1.6));
#17146=CARTESIAN_POINT('Origin',(5.8,0.,1.6));
#17147=CARTESIAN_POINT('',(5.5,1.6,1.6));
#17148=CARTESIAN_POINT('Origin',(5.5,3.2,0.));
#17149=CARTESIAN_POINT('',(5.5,3.2,0.));
#17150=CARTESIAN_POINT('',(5.5,3.2,0.));
#17151=CARTESIAN_POINT('',(5.5,3.2,0.));
#17152=CARTESIAN_POINT('',(5.5,-3.2,0.));
#17153=CARTESIAN_POINT('',(5.5,3.2,0.));
#17154=CARTESIAN_POINT('',(5.5,-3.2,0.));
#17155=CARTESIAN_POINT('Origin',(5.8,0.,0.));
#17156=CARTESIAN_POINT('',(5.5,-3.2,0.));
#17157=CARTESIAN_POINT('Origin',(5.8,0.,0.));
#17158=CARTESIAN_POINT('',(6.1,3.2,0.));
#17159=CARTESIAN_POINT('Origin',(6.1,3.2,0.));
#17160=CARTESIAN_POINT('Origin',(5.5,-3.2,0.));
#20003=UNCERTAINTY_MEASURE_WITH_UNIT(LENGTH_MEASURE(0.001),#20097,
'DISTANCE_ACCURACY_VALUE',
'Maximum model space distance between geometric entities at asserted c
onnectivities');
#20042=UNCERTAINTY_MEASURE_WITH_UNIT(LENGTH_MEASURE(0.001),#20097,
'DISTANCE_ACCURACY_VALUE',
'Maximum model space distance between geometric entities at asserted c
onnectivities');
#20057=(
GEOMETRIC_REPRESENTATION_CONTEXT(3)
GLOBAL_UNCERTAINTY_ASSIGNED_CONTEXT((#20003))
GLOBAL_UNIT_ASSIGNED_CONTEXT((#20097,#20099,#20100))
REPRESENTATION_CONTEXT('','3D')
);
#20096=(
GEOMETRIC_REPRESENTATION_CONTEXT(3)
GLOBAL_UNCERTAINTY_ASSIGNED_CONTEXT((#20042))
GLOBAL_UNIT_ASSIGNED_CONTEXT((#20097,#20099,#20100))
REPRESENTATION_CONTEXT('','3D')
);
#20097=(
LENGTH_UNIT()
NAMED_UNIT(*)
SI_UNIT(.CENTI.,.METRE.)
);
#20099=(
NAMED_UNIT(*)
PLANE_ANGLE_UNIT()
SI_UNIT($,.RADIAN.)
);
#20100=(
NAMED_UNIT(*)
SI_UNIT($,.STERADIAN.)
SOLID_ANGLE_UNIT()
);
#20115=SHAPE_DEFINITION_REPRESENTATION(#20168,#20326);
#20168=PRODUCT_DEFINITION_SHAPE('',$,#20380);
#20326=SHAPE_REPRESENTATION('',(#11850),#20057);
#20365=PRODUCT_DEFINITION_CONTEXT('part definition',#20526,'design');
#20380=PRODUCT_DEFINITION('Travel stop','Travel stop',#20433,#20365);
#20433=PRODUCT_DEFINITION_FORMATION('',$,#20542);
#20526=APPLICATION_CONTEXT(
'Core Data for Automotive Mechanical Design Process');
#20527=PRODUCT_CONTEXT('part definition',#20526,'mechanical');
#20542=PRODUCT('Travel stop','Travel stop','Travel stop',(#20527));
#20630=COLOUR_RGB('Light Blue',0.38,0.62,0.78);
#20631=FILL_AREA_STYLE_COLOUR('',#20630);
#20632=FILL_AREA_STYLE('',(#20631));
#20633=SURFACE_STYLE_FILL_AREA(#20632);
#20634=SURFACE_SIDE_STYLE('',(#20633));
#20635=SURFACE_STYLE_USAGE(.BOTH.,#20634);
#20636=PRESENTATION_STYLE_ASSIGNMENT((#20635));
ENDSEC;
END-ISO-10303-21;
